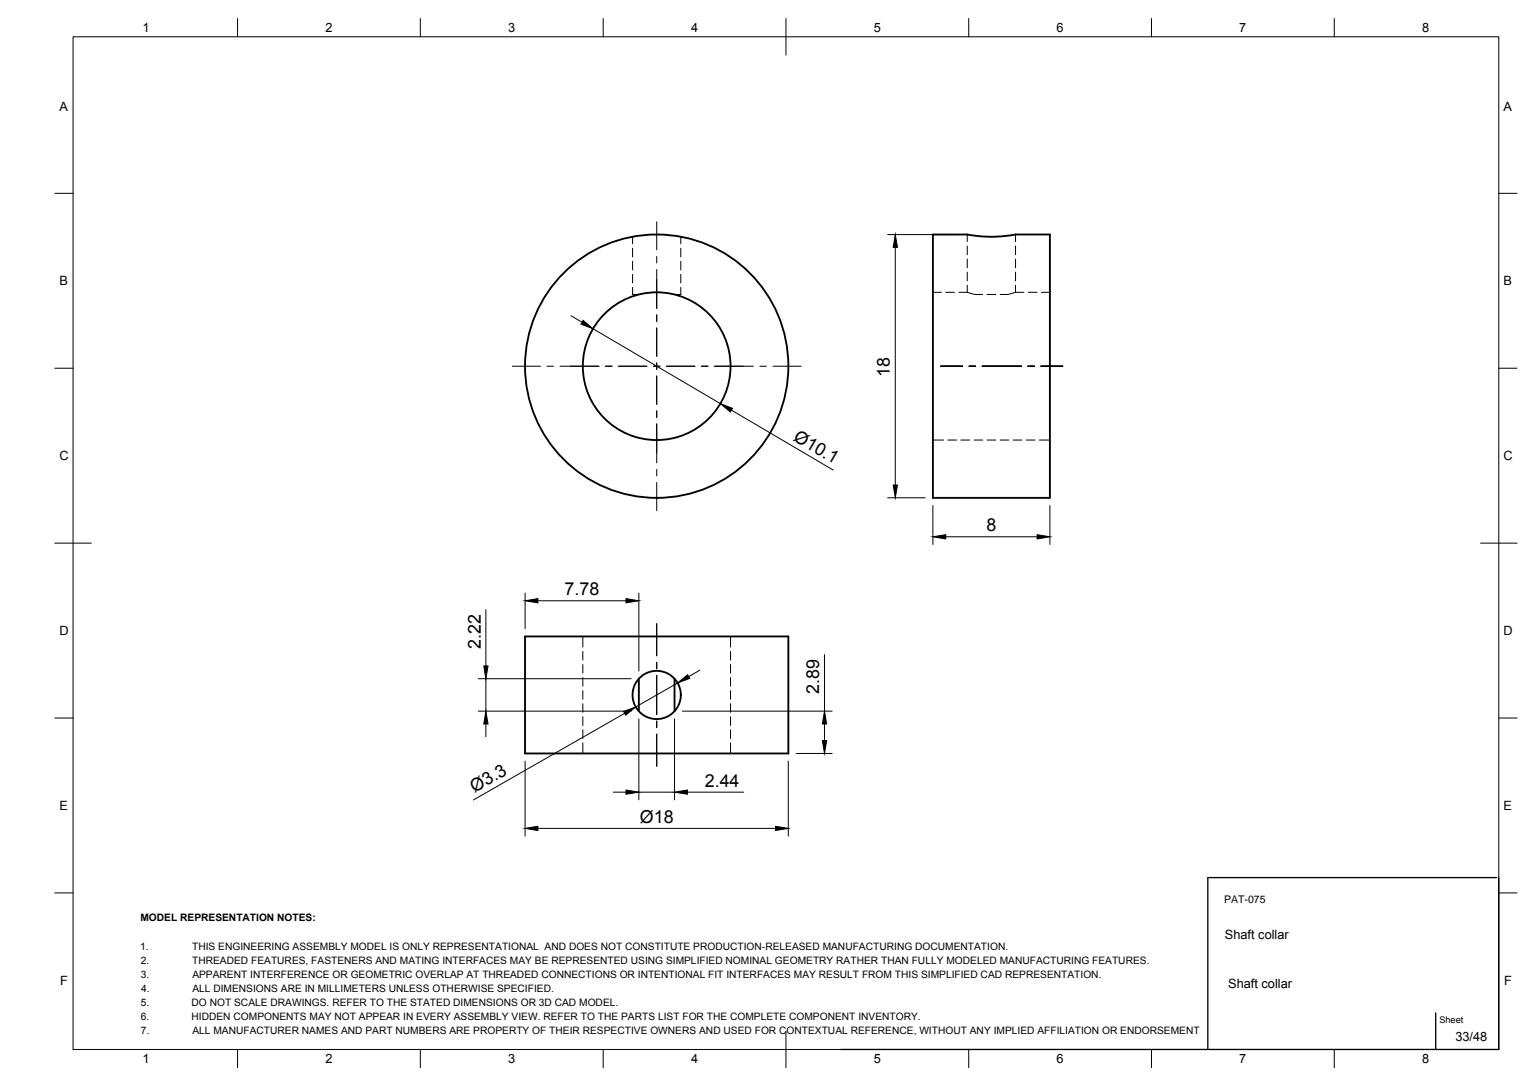
ISO-10303-21;
HEADER;
/* Generated by software containing ST-Developer
 * from STEP Tools, Inc. (www.steptools.com) 
 */

FILE_DESCRIPTION(
/* description */ ('Over-Centre Plunger Toggle Clamp on Slotted Fixture Frame'),
/* implementation_level */ '2;1');

FILE_NAME(
/* name */ 
'Shaft collar.step',
/* time_stamp */ '2026-10-28T03:23:24-07:00',
/* author */ (''),
/* organization */ (''),
/* preprocessor_version */ 'ST-DEVELOPER v20.2',
/* originating_system */ 'Autodesk Translation Framework v15.17.0.0',
/* authorisation */ '');

FILE_SCHEMA (('AUTOMOTIVE_DESIGN { 1 0 10303 214 3 1 1 }'));
ENDSEC;

DATA;
#10=MECHANICAL_DESIGN_GEOMETRIC_PRESENTATION_REPRESENTATION('',(#547),#15212);
#373=B_SPLINE_CURVE_WITH_KNOTS('',3,(#14378,#14379,#14380,#14381,#14382,
#14383,#14384,#14385,#14386,#14387,#14388,#14389,#14390,#14391),
 .UNSPECIFIED.,.F.,.F.,(4,2,2,2,2,2,4),(0.618551524396288,0.626563103102763,
0.689203386094986,0.751843669087208,0.814483952079431,0.877124235071654,
0.88513581377813),.UNSPECIFIED.);
#374=B_SPLINE_CURVE_WITH_KNOTS('',3,(#14397,#14398,#14399,#14400,#14401,
#14402,#14403,#14404,#14405,#14406,#14407,#14408,#14409,#14410,#14411,#14412,
#14413,#14414),.UNSPECIFIED.,.F.,.F.,(4,2,2,2,2,2,2,2,4),(0.,0.0623062782223138,
0.124612556444628,0.186916384615148,0.249220212785668,0.311524040956189,
0.373827869126709,0.436134147349023,0.498440425571337),.UNSPECIFIED.);
#375=B_SPLINE_CURVE_WITH_KNOTS('',3,(#14415,#14416,#14417,#14418,#14419,
#14420,#14421,#14422,#14423,#14424,#14425,#14426,#14427,#14428,#14429,#14430,
#14431,#14432),.UNSPECIFIED.,.F.,.F.,(4,2,2,2,2,2,2,2,4),(0.498440425571337,
0.560746703793651,0.623052982015964,0.685356810186485,0.747660638357005,
0.809964466527525,0.872268294698046,0.93457457292036,0.996880851142673),
 .UNSPECIFIED.);
#376=B_SPLINE_CURVE_WITH_KNOTS('',3,(#14435,#14436,#14437,#14438,#14439,
#14440,#14441,#14442,#14443,#14444,#14445,#14446,#14447,#14448),
 .UNSPECIFIED.,.F.,.F.,(4,2,2,2,2,2,4),(0.117322411671483,0.125333990377957,
0.18797427337018,0.250614556362403,0.313254839354626,0.375895122346849,
0.383906701053325),.UNSPECIFIED.);
#455=SHAPE_REPRESENTATION_RELATIONSHIP('SRR','None',#15432,#497);
#497=ADVANCED_BREP_SHAPE_REPRESENTATION('',(#596),#15194);
#547=STYLED_ITEM('',(#15719),#596);
#596=MANIFOLD_SOLID_BREP('Body1',#8281);
#749=FACE_BOUND('',#2063,.T.);
#750=FACE_BOUND('',#2065,.T.);
#751=FACE_BOUND('',#2067,.T.);
#752=FACE_BOUND('',#2069,.T.);
#997=PLANE('',#9428);
#998=PLANE('',#9433);
#999=PLANE('',#9440);
#1000=PLANE('',#9441);
#1435=FACE_OUTER_BOUND('',#2059,.T.);
#1436=FACE_OUTER_BOUND('',#2060,.T.);
#1437=FACE_OUTER_BOUND('',#2061,.T.);
#1438=FACE_OUTER_BOUND('',#2062,.T.);
#1439=FACE_OUTER_BOUND('',#2064,.T.);
#1440=FACE_OUTER_BOUND('',#2066,.T.);
#1441=FACE_OUTER_BOUND('',#2068,.T.);
#2059=EDGE_LOOP('',(#7097,#7098));
#2060=EDGE_LOOP('',(#7099,#7100,#7101,#7102,#7103,#7104,#7105,#7106,#7107));
#2061=EDGE_LOOP('',(#7108,#7109,#7110));
#2062=EDGE_LOOP('',(#7111,#7112,#7113,#7114));
#2063=EDGE_LOOP('',(#7115,#7116,#7117,#7118));
#2064=EDGE_LOOP('',(#7119,#7120,#7121,#7122));
#2065=EDGE_LOOP('',(#7123,#7124));
#2066=EDGE_LOOP('',(#7125));
#2067=EDGE_LOOP('',(#7126));
#2068=EDGE_LOOP('',(#7127));
#2069=EDGE_LOOP('',(#7128));
#2699=LINE('',#14374,#3329);
#2700=LINE('',#14395,#3330);
#2701=LINE('',#14450,#3331);
#2702=LINE('',#14455,#3332);
#2703=LINE('',#14461,#3333);
#3329=VECTOR('',#11554,1.);
#3330=VECTOR('',#11561,0.164999999999999);
#3331=VECTOR('',#11566,1.);
#3332=VECTOR('',#11571,0.505);
#3333=VECTOR('',#11578,0.9);
#3767=CIRCLE('',#9429,0.164999999999999);
#3768=CIRCLE('',#9431,0.164999999999999);
#3769=CIRCLE('',#9432,0.164999999999999);
#3770=CIRCLE('',#9435,0.505);
#3771=CIRCLE('',#9436,0.505);
#3772=CIRCLE('',#9438,0.9);
#3773=CIRCLE('',#9439,0.9);
#4375=VERTEX_POINT('',#14372);
#4376=VERTEX_POINT('',#14373);
#4377=VERTEX_POINT('',#14377);
#4378=VERTEX_POINT('',#14392);
#4379=VERTEX_POINT('',#14394);
#4380=VERTEX_POINT('',#14396);
#4381=VERTEX_POINT('',#14433);
#4382=VERTEX_POINT('',#14452);
#4383=VERTEX_POINT('',#14454);
#4384=VERTEX_POINT('',#14458);
#4385=VERTEX_POINT('',#14460);
#5309=EDGE_CURVE('',#4375,#4376,#2699,.T.);
#5310=EDGE_CURVE('',#4375,#4376,#3767,.T.);
#5311=EDGE_CURVE('',#4377,#4375,#373,.T.);
#5312=EDGE_CURVE('',#4378,#4377,#3768,.T.);
#5313=EDGE_CURVE('',#4378,#4379,#2700,.T.);
#5314=EDGE_CURVE('',#4380,#4379,#374,.T.);
#5315=EDGE_CURVE('',#4379,#4380,#375,.T.);
#5316=EDGE_CURVE('',#4381,#4378,#3769,.T.);
#5317=EDGE_CURVE('',#4376,#4381,#376,.T.);
#5318=EDGE_CURVE('',#4381,#4377,#2701,.T.);
#5319=EDGE_CURVE('',#4382,#4382,#3770,.T.);
#5320=EDGE_CURVE('',#4382,#4383,#2702,.T.);
#5321=EDGE_CURVE('',#4383,#4383,#3771,.T.);
#5322=EDGE_CURVE('',#4384,#4384,#3772,.T.);
#5323=EDGE_CURVE('',#4384,#4385,#2703,.T.);
#5324=EDGE_CURVE('',#4385,#4385,#3773,.T.);
#7097=ORIENTED_EDGE('',*,*,#5309,.F.);
#7098=ORIENTED_EDGE('',*,*,#5310,.T.);
#7099=ORIENTED_EDGE('',*,*,#5311,.F.);
#7100=ORIENTED_EDGE('',*,*,#5312,.F.);
#7101=ORIENTED_EDGE('',*,*,#5313,.T.);
#7102=ORIENTED_EDGE('',*,*,#5314,.F.);
#7103=ORIENTED_EDGE('',*,*,#5315,.F.);
#7104=ORIENTED_EDGE('',*,*,#5313,.F.);
#7105=ORIENTED_EDGE('',*,*,#5316,.F.);
#7106=ORIENTED_EDGE('',*,*,#5317,.F.);
#7107=ORIENTED_EDGE('',*,*,#5310,.F.);
#7108=ORIENTED_EDGE('',*,*,#5318,.F.);
#7109=ORIENTED_EDGE('',*,*,#5316,.T.);
#7110=ORIENTED_EDGE('',*,*,#5312,.T.);
#7111=ORIENTED_EDGE('',*,*,#5319,.F.);
#7112=ORIENTED_EDGE('',*,*,#5320,.T.);
#7113=ORIENTED_EDGE('',*,*,#5321,.T.);
#7114=ORIENTED_EDGE('',*,*,#5320,.F.);
#7115=ORIENTED_EDGE('',*,*,#5317,.T.);
#7116=ORIENTED_EDGE('',*,*,#5318,.T.);
#7117=ORIENTED_EDGE('',*,*,#5311,.T.);
#7118=ORIENTED_EDGE('',*,*,#5309,.T.);
#7119=ORIENTED_EDGE('',*,*,#5322,.F.);
#7120=ORIENTED_EDGE('',*,*,#5323,.T.);
#7121=ORIENTED_EDGE('',*,*,#5324,.T.);
#7122=ORIENTED_EDGE('',*,*,#5323,.F.);
#7123=ORIENTED_EDGE('',*,*,#5314,.T.);
#7124=ORIENTED_EDGE('',*,*,#5315,.T.);
#7125=ORIENTED_EDGE('',*,*,#5322,.T.);
#7126=ORIENTED_EDGE('',*,*,#5319,.T.);
#7127=ORIENTED_EDGE('',*,*,#5324,.F.);
#7128=ORIENTED_EDGE('',*,*,#5321,.F.);
#7721=CYLINDRICAL_SURFACE('',#9430,0.164999999999999);
#7722=CYLINDRICAL_SURFACE('',#9434,0.505);
#7723=CYLINDRICAL_SURFACE('',#9437,0.9);
#8107=ADVANCED_FACE('',(#1435),#997,.T.);
#8108=ADVANCED_FACE('',(#1436),#7721,.F.);
#8109=ADVANCED_FACE('',(#1437),#998,.T.);
#8110=ADVANCED_FACE('',(#1438,#749),#7722,.F.);
#8111=ADVANCED_FACE('',(#1439,#750),#7723,.T.);
#8112=ADVANCED_FACE('',(#1440,#751),#999,.T.);
#8113=ADVANCED_FACE('',(#1441,#752),#1000,.F.);
#8281=CLOSED_SHELL('',(#8107,#8108,#8109,#8110,#8111,#8112,#8113));
#9427=AXIS2_PLACEMENT_3D('',#14370,#11550,#11551);
#9428=AXIS2_PLACEMENT_3D('',#14371,#11552,#11553);
#9429=AXIS2_PLACEMENT_3D('',#14375,#11555,#11556);
#9430=AXIS2_PLACEMENT_3D('',#14376,#11557,#11558);
#9431=AXIS2_PLACEMENT_3D('',#14393,#11559,#11560);
#9432=AXIS2_PLACEMENT_3D('',#14434,#11562,#11563);
#9433=AXIS2_PLACEMENT_3D('',#14449,#11564,#11565);
#9434=AXIS2_PLACEMENT_3D('',#14451,#11567,#11568);
#9435=AXIS2_PLACEMENT_3D('',#14453,#11569,#11570);
#9436=AXIS2_PLACEMENT_3D('',#14456,#11572,#11573);
#9437=AXIS2_PLACEMENT_3D('',#14457,#11574,#11575);
#9438=AXIS2_PLACEMENT_3D('',#14459,#11576,#11577);
#9439=AXIS2_PLACEMENT_3D('',#14462,#11579,#11580);
#9440=AXIS2_PLACEMENT_3D('',#14463,#11581,#11582);
#9441=AXIS2_PLACEMENT_3D('',#14464,#11583,#11584);
#11550=DIRECTION('axis',(0.,0.,1.));
#11551=DIRECTION('refdir',(1.,0.,0.));
#11552=DIRECTION('center_axis',(1.,0.,0.));
#11553=DIRECTION('ref_axis',(0.,0.,-1.));
#11554=DIRECTION('',(0.,1.,0.));
#11555=DIRECTION('center_axis',(1.,0.,0.));
#11556=DIRECTION('ref_axis',(0.,0.,-1.));
#11557=DIRECTION('center_axis',(1.,0.,0.));
#11558=DIRECTION('ref_axis',(0.,0.,-1.));
#11559=DIRECTION('center_axis',(1.,0.,0.));
#11560=DIRECTION('ref_axis',(0.,0.,-1.));
#11561=DIRECTION('',(1.,0.,0.));
#11562=DIRECTION('center_axis',(1.,0.,0.));
#11563=DIRECTION('ref_axis',(0.,0.,-1.));
#11564=DIRECTION('center_axis',(1.,0.,0.));
#11565=DIRECTION('ref_axis',(0.,0.,-1.));
#11566=DIRECTION('',(0.,-1.,0.));
#11567=DIRECTION('center_axis',(0.,1.,0.));
#11568=DIRECTION('ref_axis',(1.,0.,0.));
#11569=DIRECTION('center_axis',(0.,-1.,0.));
#11570=DIRECTION('ref_axis',(1.,0.,0.));
#11571=DIRECTION('',(0.,-1.,0.));
#11572=DIRECTION('center_axis',(0.,-1.,0.));
#11573=DIRECTION('ref_axis',(1.,0.,0.));
#11574=DIRECTION('center_axis',(0.,1.,0.));
#11575=DIRECTION('ref_axis',(1.,0.,0.));
#11576=DIRECTION('center_axis',(0.,1.,0.));
#11577=DIRECTION('ref_axis',(1.,0.,0.));
#11578=DIRECTION('',(0.,-1.,0.));
#11579=DIRECTION('center_axis',(0.,1.,0.));
#11580=DIRECTION('ref_axis',(1.,0.,0.));
#11581=DIRECTION('center_axis',(0.,1.,0.));
#11582=DIRECTION('ref_axis',(1.,0.,0.));
#11583=DIRECTION('center_axis',(0.,1.,0.));
#11584=DIRECTION('ref_axis',(1.,0.,0.));
#14370=CARTESIAN_POINT('',(0.,0.,0.));
#14371=CARTESIAN_POINT('Origin',(-3.51,1.4,11.));
#14372=CARTESIAN_POINT('',(-3.51,1.28909463493591,10.8778320827713));
#14373=CARTESIAN_POINT('',(-3.51,1.51090536506409,10.8778320827713));
#14374=CARTESIAN_POINT('',(-3.51,1.,10.8778320827713));
#14375=CARTESIAN_POINT('Origin',(-3.51,1.4,11.));
#14376=CARTESIAN_POINT('Origin',(-3.51,1.4,11.));
#14377=CARTESIAN_POINT('',(-3.51,1.28909463493591,11.1221679172287));
#14378=CARTESIAN_POINT('Ctrl Pts',(-3.51,1.28909463493591,11.1221679172287));
#14379=CARTESIAN_POINT('Ctrl Pts',(-3.50955146832001,1.28711294069536,11.1203689136263));
#14380=CARTESIAN_POINT('Ctrl Pts',(-3.50910475462832,1.28518965877367,11.1185348965652));
#14381=CARTESIAN_POINT('Ctrl Pts',(-3.50520498446835,1.2687667552278,11.1021119930194));
#14382=CARTESIAN_POINT('Ctrl Pts',(-3.50155748539241,1.25609154388858,11.0836597150224));
#14383=CARTESIAN_POINT('Ctrl Pts',(-3.49642218023894,1.23920409039234,11.0430495960472));
#14384=CARTESIAN_POINT('Ctrl Pts',(-3.495,1.235,11.0208800943307));
#14385=CARTESIAN_POINT('Ctrl Pts',(-3.495,1.235,10.9791199056693));
#14386=CARTESIAN_POINT('Ctrl Pts',(-3.49642218023894,1.23920409039234,10.9569504039528));
#14387=CARTESIAN_POINT('Ctrl Pts',(-3.50155748539241,1.25609154388858,10.9163402849776));
#14388=CARTESIAN_POINT('Ctrl Pts',(-3.50520498446835,1.2687667552278,10.8978880069806));
#14389=CARTESIAN_POINT('Ctrl Pts',(-3.50910475462832,1.28518965877367,10.8814651034348));
#14390=CARTESIAN_POINT('Ctrl Pts',(-3.50955146832001,1.28711294069536,10.8796310863737));
#14391=CARTESIAN_POINT('Ctrl Pts',(-3.51,1.28909463493591,10.8778320827713));
#14392=CARTESIAN_POINT('',(-3.51,1.4,11.165));
#14393=CARTESIAN_POINT('Origin',(-3.51,1.4,11.));
#14394=CARTESIAN_POINT('',(-3.11525427381648,1.4,11.165));
#14395=CARTESIAN_POINT('',(-3.51,1.4,11.165));
#14396=CARTESIAN_POINT('',(-3.11525427381648,1.4,10.835));
#14397=CARTESIAN_POINT('Ctrl Pts',(-3.11525427381648,1.4,10.835));
#14398=CARTESIAN_POINT('Ctrl Pts',(-3.11525427381648,1.37923124059256,10.835));
#14399=CARTESIAN_POINT('Ctrl Pts',(-3.11444724049474,1.35711110492666,10.8391602809924));
#14400=CARTESIAN_POINT('Ctrl Pts',(-3.11155135184996,1.31647293736623,10.8560135297833));
#14401=CARTESIAN_POINT('Ctrl Pts',(-3.10950639514836,1.29795075602263,10.8687040061858));
#14402=CARTESIAN_POINT('Ctrl Pts',(-3.10568276567606,1.26870458121656,10.8979501809919));
#14403=CARTESIAN_POINT('Ctrl Pts',(-3.10365291110046,1.25601365401642,10.9164726079093));
#14404=CARTESIAN_POINT('Ctrl Pts',(-3.10079172813942,1.23916007816136,10.9571116239066));
#14405=CARTESIAN_POINT('Ctrl Pts',(-3.1,1.235,10.9792320572765));
#14406=CARTESIAN_POINT('Ctrl Pts',(-3.1,1.235,11.0207679427235));
#14407=CARTESIAN_POINT('Ctrl Pts',(-3.10079172813942,1.23916007816136,11.0428883760934));
#14408=CARTESIAN_POINT('Ctrl Pts',(-3.10365291110046,1.25601365401642,11.0835273920907));
#14409=CARTESIAN_POINT('Ctrl Pts',(-3.10568276567606,1.26870458121656,11.1020498190081));
#14410=CARTESIAN_POINT('Ctrl Pts',(-3.10950639514836,1.29795075602263,11.1312959938142));
#14411=CARTESIAN_POINT('Ctrl Pts',(-3.11155135184996,1.31647293736623,11.1439864702167));
#14412=CARTESIAN_POINT('Ctrl Pts',(-3.11444724049474,1.35711110492666,11.1608397190076));
#14413=CARTESIAN_POINT('Ctrl Pts',(-3.11525427381648,1.37923124059256,11.165));
#14414=CARTESIAN_POINT('Ctrl Pts',(-3.11525427381648,1.4,11.165));
#14415=CARTESIAN_POINT('Ctrl Pts',(-3.11525427381648,1.4,11.165));
#14416=CARTESIAN_POINT('Ctrl Pts',(-3.11525427381648,1.42076875940744,11.165));
#14417=CARTESIAN_POINT('Ctrl Pts',(-3.11444724049474,1.44288889507334,11.1608397190076));
#14418=CARTESIAN_POINT('Ctrl Pts',(-3.11155135184996,1.48352706263377,11.1439864702167));
#14419=CARTESIAN_POINT('Ctrl Pts',(-3.10950639514836,1.50204924397737,11.1312959938142));
#14420=CARTESIAN_POINT('Ctrl Pts',(-3.10568276567606,1.53129541878343,11.1020498190081));
#14421=CARTESIAN_POINT('Ctrl Pts',(-3.10365291110046,1.54398634598358,11.0835273920907));
#14422=CARTESIAN_POINT('Ctrl Pts',(-3.10079172813942,1.56083992183864,11.0428883760934));
#14423=CARTESIAN_POINT('Ctrl Pts',(-3.1,1.565,11.0207679427235));
#14424=CARTESIAN_POINT('Ctrl Pts',(-3.1,1.565,10.9792320572765));
#14425=CARTESIAN_POINT('Ctrl Pts',(-3.10079172813942,1.56083992183864,10.9571116239066));
#14426=CARTESIAN_POINT('Ctrl Pts',(-3.10365291110046,1.54398634598358,10.9164726079093));
#14427=CARTESIAN_POINT('Ctrl Pts',(-3.10568276567606,1.53129541878343,10.8979501809919));
#14428=CARTESIAN_POINT('Ctrl Pts',(-3.10950639514836,1.50204924397737,10.8687040061858));
#14429=CARTESIAN_POINT('Ctrl Pts',(-3.11155135184996,1.48352706263377,10.8560135297833));
#14430=CARTESIAN_POINT('Ctrl Pts',(-3.11444724049474,1.44288889507334,10.8391602809924));
#14431=CARTESIAN_POINT('Ctrl Pts',(-3.11525427381648,1.42076875940744,10.835));
#14432=CARTESIAN_POINT('Ctrl Pts',(-3.11525427381648,1.4,10.835));
#14433=CARTESIAN_POINT('',(-3.51,1.51090536506409,11.1221679172287));
#14434=CARTESIAN_POINT('Origin',(-3.51,1.4,11.));
#14435=CARTESIAN_POINT('Ctrl Pts',(-3.51,1.51090536506409,10.8778320827713));
#14436=CARTESIAN_POINT('Ctrl Pts',(-3.50955146832001,1.51288705930464,10.8796310863737));
#14437=CARTESIAN_POINT('Ctrl Pts',(-3.50910475462832,1.51481034122633,10.8814651034348));
#14438=CARTESIAN_POINT('Ctrl Pts',(-3.50520498446835,1.5312332447722,10.8978880069806));
#14439=CARTESIAN_POINT('Ctrl Pts',(-3.50155748539241,1.54390845611142,10.9163402849776));
#14440=CARTESIAN_POINT('Ctrl Pts',(-3.49642218023894,1.56079590960766,10.9569504039528));
#14441=CARTESIAN_POINT('Ctrl Pts',(-3.495,1.565,10.9791199056693));
#14442=CARTESIAN_POINT('Ctrl Pts',(-3.495,1.565,11.0208800943307));
#14443=CARTESIAN_POINT('Ctrl Pts',(-3.49642218023894,1.56079590960766,11.0430495960472));
#14444=CARTESIAN_POINT('Ctrl Pts',(-3.50155748539241,1.54390845611142,11.0836597150224));
#14445=CARTESIAN_POINT('Ctrl Pts',(-3.50520498446835,1.5312332447722,11.1021119930194));
#14446=CARTESIAN_POINT('Ctrl Pts',(-3.50910475462832,1.51481034122633,11.1185348965652));
#14447=CARTESIAN_POINT('Ctrl Pts',(-3.50955146832001,1.51288705930464,11.1203689136263));
#14448=CARTESIAN_POINT('Ctrl Pts',(-3.51,1.51090536506409,11.1221679172287));
#14449=CARTESIAN_POINT('Origin',(-3.51,1.4,11.));
#14450=CARTESIAN_POINT('',(-3.51,1.,11.1221679172287));
#14451=CARTESIAN_POINT('Origin',(-4.,1.,11.));
#14452=CARTESIAN_POINT('',(-4.505,1.8,11.));
#14453=CARTESIAN_POINT('Origin',(-4.,1.8,11.));
#14454=CARTESIAN_POINT('',(-4.505,1.,11.));
#14455=CARTESIAN_POINT('',(-4.505,1.,11.));
#14456=CARTESIAN_POINT('Origin',(-4.,1.,11.));
#14457=CARTESIAN_POINT('Origin',(-4.,1.,11.));
#14458=CARTESIAN_POINT('',(-4.9,1.8,11.));
#14459=CARTESIAN_POINT('Origin',(-4.,1.8,11.));
#14460=CARTESIAN_POINT('',(-4.9,1.,11.));
#14461=CARTESIAN_POINT('',(-4.9,1.,11.));
#14462=CARTESIAN_POINT('Origin',(-4.,1.,11.));
#14463=CARTESIAN_POINT('Origin',(-4.,1.8,11.));
#14464=CARTESIAN_POINT('Origin',(-4.,1.,11.));
#15144=UNCERTAINTY_MEASURE_WITH_UNIT(LENGTH_MEASURE(0.001),#15213,
'DISTANCE_ACCURACY_VALUE',
'Maximum model space distance between geometric entities at asserted c
onnectivities');
#15162=UNCERTAINTY_MEASURE_WITH_UNIT(LENGTH_MEASURE(0.001),#15213,
'DISTANCE_ACCURACY_VALUE',
'Maximum model space distance between geometric entities at asserted c
onnectivities');
#15194=(
GEOMETRIC_REPRESENTATION_CONTEXT(3)
GLOBAL_UNCERTAINTY_ASSIGNED_CONTEXT((#15144))
GLOBAL_UNIT_ASSIGNED_CONTEXT((#15213,#15215,#15216))
REPRESENTATION_CONTEXT('','3D')
);
#15212=(
GEOMETRIC_REPRESENTATION_CONTEXT(3)
GLOBAL_UNCERTAINTY_ASSIGNED_CONTEXT((#15162))
GLOBAL_UNIT_ASSIGNED_CONTEXT((#15213,#15215,#15216))
REPRESENTATION_CONTEXT('','3D')
);
#15213=(
LENGTH_UNIT()
NAMED_UNIT(*)
SI_UNIT(.CENTI.,.METRE.)
);
#15215=(
NAMED_UNIT(*)
PLANE_ANGLE_UNIT()
SI_UNIT($,.RADIAN.)
);
#15216=(
NAMED_UNIT(*)
SI_UNIT($,.STERADIAN.)
SOLID_ANGLE_UNIT()
);
#15248=SHAPE_DEFINITION_REPRESENTATION(#15304,#15432);
#15304=PRODUCT_DEFINITION_SHAPE('',$,#15482);
#15432=SHAPE_REPRESENTATION('',(#9427),#15194);
#15450=PRODUCT_DEFINITION_CONTEXT('part definition',#15599,'design');
#15482=PRODUCT_DEFINITION('Shaft collar','Shaft collar',#15531,#15450);
#15531=PRODUCT_DEFINITION_FORMATION('',$,#15632);
#15599=APPLICATION_CONTEXT(
'Core Data for Automotive Mechanical Design Process');
#15600=PRODUCT_CONTEXT('part definition',#15599,'mechanical');
#15632=PRODUCT('Shaft collar','Shaft collar','Shaft collar',(#15600));
#15713=COLOUR_RGB('Grey',0.48,0.52,0.57);
#15714=FILL_AREA_STYLE_COLOUR('',#15713);
#15715=FILL_AREA_STYLE('',(#15714));
#15716=SURFACE_STYLE_FILL_AREA(#15715);
#15717=SURFACE_SIDE_STYLE('',(#15716));
#15718=SURFACE_STYLE_USAGE(.BOTH.,#15717);
#15719=PRESENTATION_STYLE_ASSIGNMENT((#15718));
ENDSEC;
END-ISO-10303-21;
